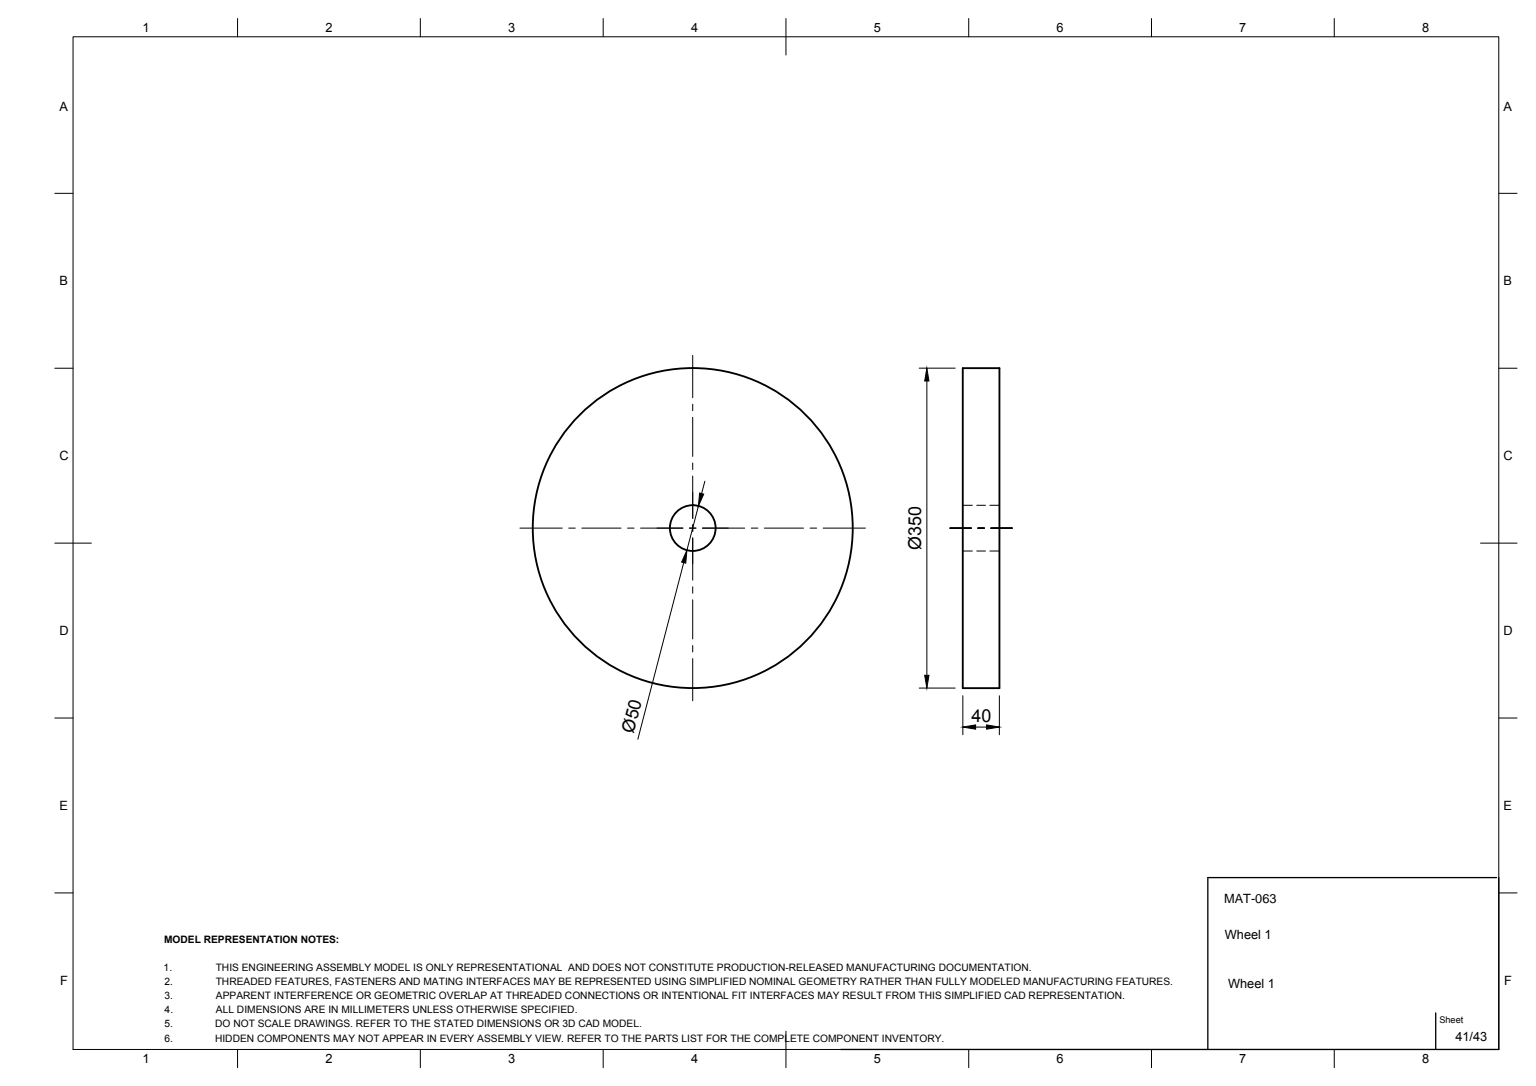
ISO-10303-21;
HEADER;
/* Generated by software containing ST-Developer
 * from STEP Tools, Inc. (www.steptools.com) 
 */

FILE_DESCRIPTION(
/* description */ (''),
/* implementation_level */ '2;1');

FILE_NAME(
/* name */ 'Wheel 1.step',
/* time_stamp */ '2026-10-24T09:43:01-07:00',
/* author */ (''),
/* organization */ (''),
/* preprocessor_version */ 'ST-DEVELOPER v20.2',
/* originating_system */ 'Autodesk Translation Framework v15.15.0.0',
/* authorisation */ '');

FILE_SCHEMA (('AUTOMOTIVE_DESIGN { 1 0 10303 214 3 1 1 }'));
ENDSEC;

DATA;
#10=MECHANICAL_DESIGN_GEOMETRIC_PRESENTATION_REPRESENTATION('',(#303),#11112);
#237=SHAPE_REPRESENTATION_RELATIONSHIP('SRR','None',#11264,#270);
#270=ADVANCED_BREP_SHAPE_REPRESENTATION('',(#336),#11109);
#303=STYLED_ITEM('',(#11426),#336);
#336=MANIFOLD_SOLID_BREP('Wheel 1',#6040);
#492=FACE_BOUND('',#1545,.T.);
#493=FACE_BOUND('',#1547,.T.);
#659=PLANE('',#7221);
#660=PLANE('',#7223);
#1026=FACE_OUTER_BOUND('',#1543,.T.);
#1027=FACE_OUTER_BOUND('',#1544,.T.);
#1028=FACE_OUTER_BOUND('',#1546,.T.);
#1029=FACE_OUTER_BOUND('',#1548,.T.);
#1543=EDGE_LOOP('',(#5469,#5470,#5471,#5472));
#1544=EDGE_LOOP('',(#5473));
#1545=EDGE_LOOP('',(#5474));
#1546=EDGE_LOOP('',(#5475));
#1547=EDGE_LOOP('',(#5476));
#1548=EDGE_LOOP('',(#5477,#5478,#5479,#5480));
#1912=LINE('',#10982,#2271);
#1913=LINE('',#10991,#2272);
#2271=VECTOR('',#9240,0.025);
#2272=VECTOR('',#9253,0.174999999);
#2672=CIRCLE('',#7219,0.025);
#2673=CIRCLE('',#7220,0.025);
#2674=CIRCLE('',#7222,0.174999999);
#2675=CIRCLE('',#7224,0.174999999);
#3170=VERTEX_POINT('',#10979);
#3171=VERTEX_POINT('',#10981);
#3172=VERTEX_POINT('',#10985);
#3173=VERTEX_POINT('',#10988);
#3938=EDGE_CURVE('',#3170,#3170,#2672,.T.);
#3939=EDGE_CURVE('',#3170,#3171,#1912,.T.);
#3940=EDGE_CURVE('',#3171,#3171,#2673,.F.);
#3941=EDGE_CURVE('',#3172,#3172,#2674,.F.);
#3942=EDGE_CURVE('',#3173,#3173,#2675,.F.);
#3943=EDGE_CURVE('',#3172,#3173,#1913,.T.);
#5469=ORIENTED_EDGE('',*,*,#3938,.F.);
#5470=ORIENTED_EDGE('',*,*,#3939,.T.);
#5471=ORIENTED_EDGE('',*,*,#3940,.F.);
#5472=ORIENTED_EDGE('',*,*,#3939,.F.);
#5473=ORIENTED_EDGE('',*,*,#3941,.F.);
#5474=ORIENTED_EDGE('',*,*,#3940,.T.);
#5475=ORIENTED_EDGE('',*,*,#3942,.T.);
#5476=ORIENTED_EDGE('',*,*,#3938,.T.);
#5477=ORIENTED_EDGE('',*,*,#3941,.T.);
#5478=ORIENTED_EDGE('',*,*,#3943,.T.);
#5479=ORIENTED_EDGE('',*,*,#3942,.F.);
#5480=ORIENTED_EDGE('',*,*,#3943,.F.);
#5641=CYLINDRICAL_SURFACE('',#7218,0.025);
#5642=CYLINDRICAL_SURFACE('',#7225,0.174999999);
#5999=ADVANCED_FACE('',(#1026),#5641,.F.);
#6000=ADVANCED_FACE('',(#1027,#492),#659,.F.);
#6001=ADVANCED_FACE('',(#1028,#493),#660,.T.);
#6002=ADVANCED_FACE('',(#1029),#5642,.T.);
#6040=CLOSED_SHELL('',(#5999,#6000,#6001,#6002));
#7217=AXIS2_PLACEMENT_3D('',#10977,#9234,#9235);
#7218=AXIS2_PLACEMENT_3D('',#10978,#9236,#9237);
#7219=AXIS2_PLACEMENT_3D('',#10980,#9238,#9239);
#7220=AXIS2_PLACEMENT_3D('',#10983,#9241,#9242);
#7221=AXIS2_PLACEMENT_3D('',#10984,#9243,#9244);
#7222=AXIS2_PLACEMENT_3D('',#10986,#9245,#9246);
#7223=AXIS2_PLACEMENT_3D('',#10987,#9247,#9248);
#7224=AXIS2_PLACEMENT_3D('',#10989,#9249,#9250);
#7225=AXIS2_PLACEMENT_3D('',#10990,#9251,#9252);
#9234=DIRECTION('axis',(0.,0.,1.));
#9235=DIRECTION('refdir',(1.,0.,0.));
#9236=DIRECTION('center_axis',(-1.,0.,0.));
#9237=DIRECTION('ref_axis',(0.,0.,1.));
#9238=DIRECTION('center_axis',(-1.,0.,0.));
#9239=DIRECTION('ref_axis',(0.,0.,1.));
#9240=DIRECTION('',(-1.,0.,0.));
#9241=DIRECTION('center_axis',(-1.,0.,0.));
#9242=DIRECTION('ref_axis',(0.,0.,1.));
#9243=DIRECTION('center_axis',(1.,4.89404439732965E-17,-4.89404438350122E-17));
#9244=DIRECTION('ref_axis',(-4.89404439732965E-17,1.,-7.23876700762992E-50));
#9245=DIRECTION('center_axis',(-1.,0.,0.));
#9246=DIRECTION('ref_axis',(0.,0.,1.));
#9247=DIRECTION('center_axis',(1.,0.,0.));
#9248=DIRECTION('ref_axis',(0.,0.,-1.));
#9249=DIRECTION('center_axis',(-1.,0.,0.));
#9250=DIRECTION('ref_axis',(0.,0.,1.));
#9251=DIRECTION('center_axis',(-1.,0.,0.));
#9252=DIRECTION('ref_axis',(0.,0.,1.));
#9253=DIRECTION('',(1.,0.,0.));
#10977=CARTESIAN_POINT('',(0.,0.,0.));
#10978=CARTESIAN_POINT('Origin',(0.595,-0.386547301,0.));
#10979=CARTESIAN_POINT('',(0.595,-0.386547301,-0.025));
#10980=CARTESIAN_POINT('Origin',(0.595,-0.386547301,0.));
#10981=CARTESIAN_POINT('',(0.555,-0.386547301,-0.025));
#10982=CARTESIAN_POINT('',(0.595,-0.386547301,-0.025));
#10983=CARTESIAN_POINT('Origin',(0.555,-0.386547301,0.));
#10984=CARTESIAN_POINT('Origin',(0.555,-0.3865473015,4.16333634234433E-19));
#10985=CARTESIAN_POINT('',(0.555,-0.386547301,-0.174999999));
#10986=CARTESIAN_POINT('Origin',(0.555,-0.386547301,0.));
#10987=CARTESIAN_POINT('Origin',(0.595,-0.3865473015,4.16333634234433E-19));
#10988=CARTESIAN_POINT('',(0.595,-0.386547301,-0.174999999));
#10989=CARTESIAN_POINT('Origin',(0.595,-0.386547301,0.));
#10990=CARTESIAN_POINT('Origin',(0.595,-0.386547301,0.));
#10991=CARTESIAN_POINT('',(0.595,-0.386547301,-0.174999999));
#11070=UNCERTAINTY_MEASURE_WITH_UNIT(LENGTH_MEASURE(1.E-5),#11113,
'DISTANCE_ACCURACY_VALUE',
'Maximum model space distance between geometric entities at asserted c
onnectivities');
#11073=UNCERTAINTY_MEASURE_WITH_UNIT(LENGTH_MEASURE(1.E-5),#11113,
'DISTANCE_ACCURACY_VALUE',
'Maximum model space distance between geometric entities at asserted c
onnectivities');
#11109=(
GEOMETRIC_REPRESENTATION_CONTEXT(3)
GLOBAL_UNCERTAINTY_ASSIGNED_CONTEXT((#11070))
GLOBAL_UNIT_ASSIGNED_CONTEXT((#11113,#11114,#11115))
REPRESENTATION_CONTEXT('','3D')
);
#11112=(
GEOMETRIC_REPRESENTATION_CONTEXT(3)
GLOBAL_UNCERTAINTY_ASSIGNED_CONTEXT((#11073))
GLOBAL_UNIT_ASSIGNED_CONTEXT((#11113,#11114,#11115))
REPRESENTATION_CONTEXT('','3D')
);
#11113=(
LENGTH_UNIT()
NAMED_UNIT(*)
SI_UNIT($,.METRE.)
);
#11114=(
NAMED_UNIT(*)
PLANE_ANGLE_UNIT()
SI_UNIT($,.RADIAN.)
);
#11115=(
NAMED_UNIT(*)
SI_UNIT($,.STERADIAN.)
SOLID_ANGLE_UNIT()
);
#11151=SHAPE_DEFINITION_REPRESENTATION(#11207,#11264);
#11207=PRODUCT_DEFINITION_SHAPE('',$,#11303);
#11264=SHAPE_REPRESENTATION('',(#7217),#11109);
#11267=PRODUCT_DEFINITION_CONTEXT('part definition',#11383,'design');
#11303=PRODUCT_DEFINITION('Wheel 1','Wheel 1',#11341,#11267);
#11341=PRODUCT_DEFINITION_FORMATION('',$,#11420);
#11383=APPLICATION_CONTEXT(
'Core Data for Automotive Mechanical Design Process');
#11384=PRODUCT_CONTEXT('part definition',#11383,'mechanical');
#11420=PRODUCT('Wheel 1','Wheel 1','wheel__ DE     9941',(#11384));
#11426=PRESENTATION_STYLE_ASSIGNMENT((#11430));
#11430=SURFACE_STYLE_USAGE(.BOTH.,#11434);
#11434=SURFACE_SIDE_STYLE('',(#11438));
#11438=SURFACE_STYLE_FILL_AREA(#11442);
#11442=FILL_AREA_STYLE('Opaque(202,209,238)',(#11446));
#11446=FILL_AREA_STYLE_COLOUR('Opaque(202,209,238)',#11450);
#11450=COLOUR_RGB('Opaque(202,209,238)',0.792156862745098,0.819607843137255,
0.933333333333333);
ENDSEC;
END-ISO-10303-21;
